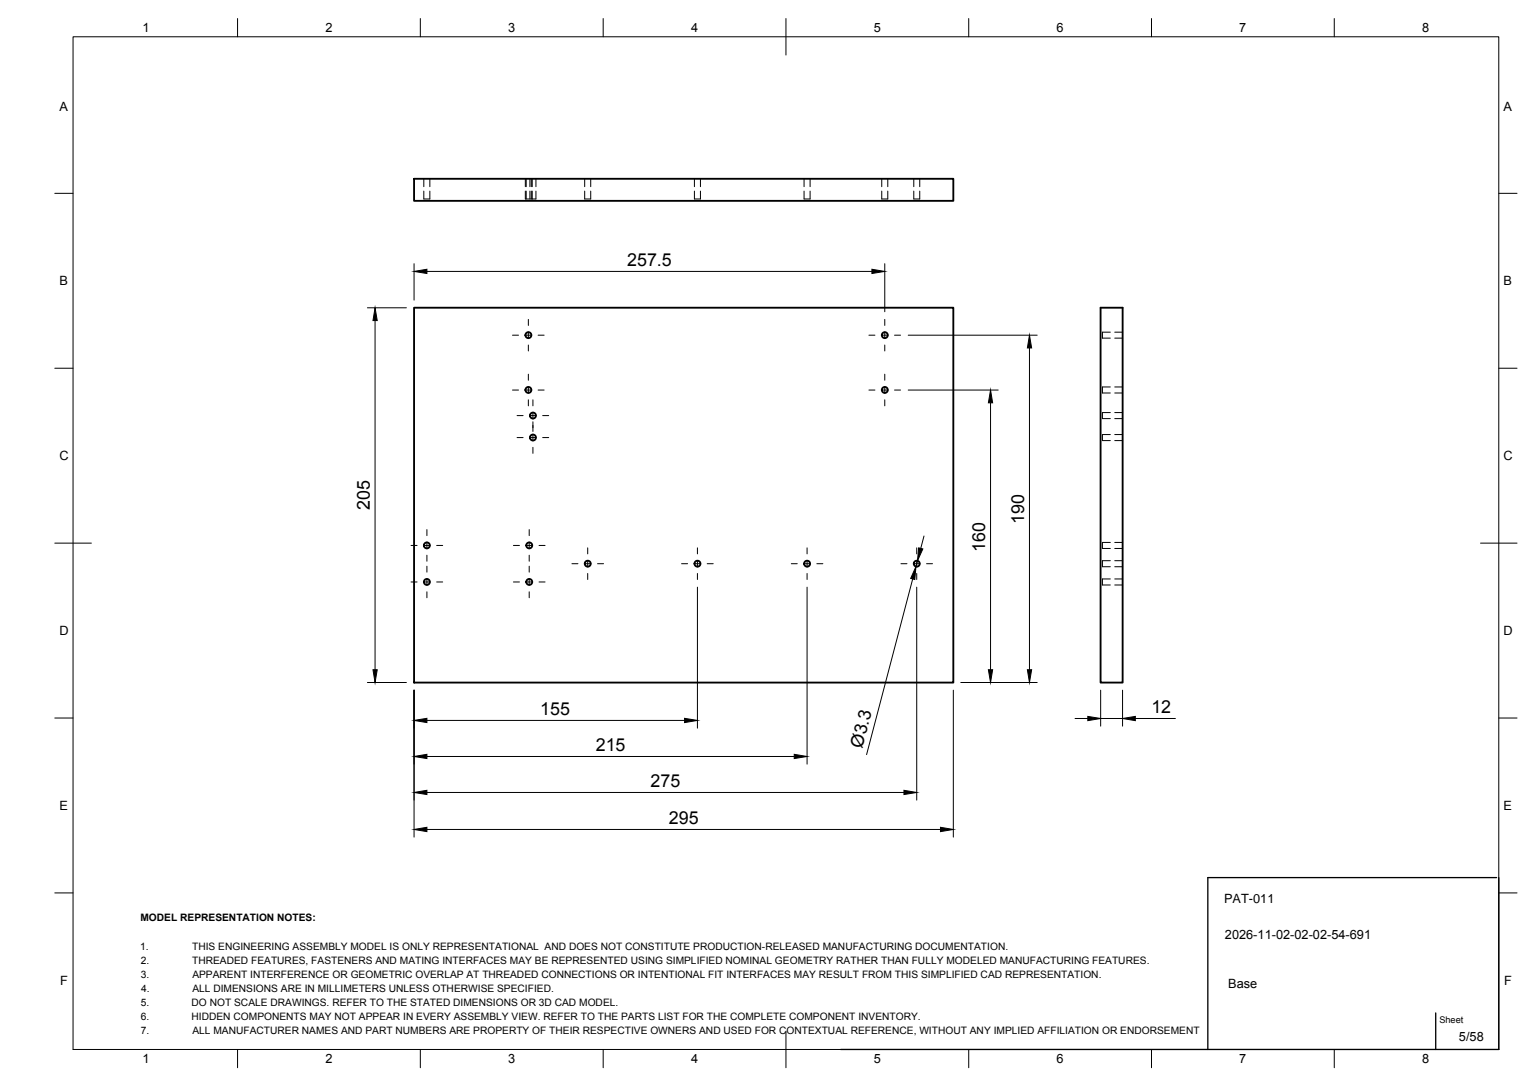
ISO-10303-21;
HEADER;
/* Generated by software containing ST-Developer
 * from STEP Tools, Inc. (www.steptools.com) 
 */

FILE_DESCRIPTION(
/* description */ ('Belt tension measurement rig'),
/* implementation_level */ '2;1');

FILE_NAME(
/* name */ 'Base.step',
/* time_stamp */ '2026-10-28T03:24:44-07:00',
/* author */ (''),
/* organization */ (''),
/* preprocessor_version */ 'ST-DEVELOPER v20.2',
/* originating_system */ 'Autodesk Translation Framework v15.17.0.0',
/* authorisation */ '');

FILE_SCHEMA (('AUTOMOTIVE_DESIGN { 1 0 10303 214 3 1 1 }'));
ENDSEC;

DATA;
#10=MECHANICAL_DESIGN_GEOMETRIC_PRESENTATION_REPRESENTATION('',(#692),#23587);
#582=SHAPE_REPRESENTATION_RELATIONSHIP('SRR','None',#23827,#637);
#637=ADVANCED_BREP_SHAPE_REPRESENTATION('',(#762),#23525);
#692=STYLED_ITEM('',(#24190),#762);
#762=MANIFOLD_SOLID_BREP('Body1',#12197);
#829=FACE_BOUND('',#2089,.T.);
#830=FACE_BOUND('',#2090,.T.);
#831=FACE_BOUND('',#2091,.T.);
#832=FACE_BOUND('',#2092,.T.);
#833=FACE_BOUND('',#2093,.T.);
#834=FACE_BOUND('',#2094,.T.);
#835=FACE_BOUND('',#2095,.T.);
#836=FACE_BOUND('',#2096,.T.);
#837=FACE_BOUND('',#2097,.T.);
#838=FACE_BOUND('',#2098,.T.);
#839=FACE_BOUND('',#2099,.T.);
#840=FACE_BOUND('',#2100,.T.);
#841=FACE_BOUND('',#2101,.T.);
#842=FACE_BOUND('',#2102,.T.);
#1037=PLANE('',#12882);
#1038=PLANE('',#12886);
#1039=PLANE('',#12890);
#1040=PLANE('',#12894);
#1041=PLANE('',#12898);
#1042=PLANE('',#12902);
#1043=PLANE('',#12906);
#1044=PLANE('',#12910);
#1045=PLANE('',#12914);
#1046=PLANE('',#12918);
#1047=PLANE('',#12922);
#1048=PLANE('',#12926);
#1049=PLANE('',#12930);
#1050=PLANE('',#12934);
#1051=PLANE('',#12935);
#1052=PLANE('',#12936);
#1053=PLANE('',#12937);
#1054=PLANE('',#12938);
#1055=PLANE('',#12939);
#1056=PLANE('',#12940);
#1352=FACE_OUTER_BOUND('',#2056,.T.);
#1353=FACE_OUTER_BOUND('',#2057,.T.);
#1354=FACE_OUTER_BOUND('',#2058,.T.);
#1355=FACE_OUTER_BOUND('',#2059,.T.);
#1356=FACE_OUTER_BOUND('',#2060,.T.);
#1357=FACE_OUTER_BOUND('',#2061,.T.);
#1358=FACE_OUTER_BOUND('',#2062,.T.);
#1359=FACE_OUTER_BOUND('',#2063,.T.);
#1360=FACE_OUTER_BOUND('',#2064,.T.);
#1361=FACE_OUTER_BOUND('',#2065,.T.);
#1362=FACE_OUTER_BOUND('',#2066,.T.);
#1363=FACE_OUTER_BOUND('',#2067,.T.);
#1364=FACE_OUTER_BOUND('',#2068,.T.);
#1365=FACE_OUTER_BOUND('',#2069,.T.);
#1366=FACE_OUTER_BOUND('',#2070,.T.);
#1367=FACE_OUTER_BOUND('',#2071,.T.);
#1368=FACE_OUTER_BOUND('',#2072,.T.);
#1369=FACE_OUTER_BOUND('',#2073,.T.);
#1370=FACE_OUTER_BOUND('',#2074,.T.);
#1371=FACE_OUTER_BOUND('',#2075,.T.);
#1372=FACE_OUTER_BOUND('',#2076,.T.);
#1373=FACE_OUTER_BOUND('',#2077,.T.);
#1374=FACE_OUTER_BOUND('',#2078,.T.);
#1375=FACE_OUTER_BOUND('',#2079,.T.);
#1376=FACE_OUTER_BOUND('',#2080,.T.);
#1377=FACE_OUTER_BOUND('',#2081,.T.);
#1378=FACE_OUTER_BOUND('',#2082,.T.);
#1379=FACE_OUTER_BOUND('',#2083,.T.);
#1380=FACE_OUTER_BOUND('',#2084,.T.);
#1381=FACE_OUTER_BOUND('',#2085,.T.);
#1382=FACE_OUTER_BOUND('',#2086,.T.);
#1383=FACE_OUTER_BOUND('',#2087,.T.);
#1384=FACE_OUTER_BOUND('',#2088,.T.);
#1385=FACE_OUTER_BOUND('',#2103,.T.);
#2056=EDGE_LOOP('',(#7938,#7939,#7940,#7941));
#2057=EDGE_LOOP('',(#7942));
#2058=EDGE_LOOP('',(#7943,#7944,#7945,#7946));
#2059=EDGE_LOOP('',(#7947));
#2060=EDGE_LOOP('',(#7948,#7949,#7950,#7951));
#2061=EDGE_LOOP('',(#7952));
#2062=EDGE_LOOP('',(#7953,#7954,#7955,#7956));
#2063=EDGE_LOOP('',(#7957));
#2064=EDGE_LOOP('',(#7958,#7959,#7960,#7961));
#2065=EDGE_LOOP('',(#7962));
#2066=EDGE_LOOP('',(#7963,#7964,#7965,#7966));
#2067=EDGE_LOOP('',(#7967));
#2068=EDGE_LOOP('',(#7968,#7969,#7970,#7971));
#2069=EDGE_LOOP('',(#7972));
#2070=EDGE_LOOP('',(#7973,#7974,#7975,#7976));
#2071=EDGE_LOOP('',(#7977));
#2072=EDGE_LOOP('',(#7978,#7979,#7980,#7981));
#2073=EDGE_LOOP('',(#7982));
#2074=EDGE_LOOP('',(#7983,#7984,#7985,#7986));
#2075=EDGE_LOOP('',(#7987));
#2076=EDGE_LOOP('',(#7988,#7989,#7990,#7991));
#2077=EDGE_LOOP('',(#7992));
#2078=EDGE_LOOP('',(#7993,#7994,#7995,#7996));
#2079=EDGE_LOOP('',(#7997));
#2080=EDGE_LOOP('',(#7998,#7999,#8000,#8001));
#2081=EDGE_LOOP('',(#8002));
#2082=EDGE_LOOP('',(#8003,#8004,#8005,#8006));
#2083=EDGE_LOOP('',(#8007));
#2084=EDGE_LOOP('',(#8008,#8009,#8010,#8011));
#2085=EDGE_LOOP('',(#8012,#8013,#8014,#8015));
#2086=EDGE_LOOP('',(#8016,#8017,#8018,#8019));
#2087=EDGE_LOOP('',(#8020,#8021,#8022,#8023));
#2088=EDGE_LOOP('',(#8024,#8025,#8026,#8027));
#2089=EDGE_LOOP('',(#8028));
#2090=EDGE_LOOP('',(#8029));
#2091=EDGE_LOOP('',(#8030));
#2092=EDGE_LOOP('',(#8031));
#2093=EDGE_LOOP('',(#8032));
#2094=EDGE_LOOP('',(#8033));
#2095=EDGE_LOOP('',(#8034));
#2096=EDGE_LOOP('',(#8035));
#2097=EDGE_LOOP('',(#8036));
#2098=EDGE_LOOP('',(#8037));
#2099=EDGE_LOOP('',(#8038));
#2100=EDGE_LOOP('',(#8039));
#2101=EDGE_LOOP('',(#8040));
#2102=EDGE_LOOP('',(#8041));
#2103=EDGE_LOOP('',(#8042,#8043,#8044,#8045));
#2968=LINE('',#18557,#3719);
#2969=LINE('',#18564,#3720);
#2970=LINE('',#18571,#3721);
#2971=LINE('',#18578,#3722);
#2972=LINE('',#18585,#3723);
#2973=LINE('',#18592,#3724);
#2974=LINE('',#18599,#3725);
#2975=LINE('',#18606,#3726);
#2976=LINE('',#18613,#3727);
#2977=LINE('',#18620,#3728);
#2978=LINE('',#18627,#3729);
#2979=LINE('',#18634,#3730);
#2980=LINE('',#18641,#3731);
#2981=LINE('',#18648,#3732);
#2982=LINE('',#18654,#3733);
#2983=LINE('',#18656,#3734);
#2984=LINE('',#18658,#3735);
#2985=LINE('',#18659,#3736);
#2986=LINE('',#18662,#3737);
#2987=LINE('',#18664,#3738);
#2988=LINE('',#18665,#3739);
#2989=LINE('',#18668,#3740);
#2990=LINE('',#18670,#3741);
#2991=LINE('',#18671,#3742);
#2992=LINE('',#18673,#3743);
#2993=LINE('',#18674,#3744);
#3719=VECTOR('',#14527,0.165);
#3720=VECTOR('',#14536,0.165);
#3721=VECTOR('',#14545,0.164999999999999);
#3722=VECTOR('',#14554,0.164999999999999);
#3723=VECTOR('',#14563,0.165);
#3724=VECTOR('',#14572,0.165);
#3725=VECTOR('',#14581,0.165);
#3726=VECTOR('',#14590,0.165);
#3727=VECTOR('',#14599,0.165);
#3728=VECTOR('',#14608,0.165);
#3729=VECTOR('',#14617,0.164999999999999);
#3730=VECTOR('',#14626,0.164999999999999);
#3731=VECTOR('',#14635,0.165);
#3732=VECTOR('',#14644,0.164999999999999);
#3733=VECTOR('',#14651,1.);
#3734=VECTOR('',#14652,1.);
#3735=VECTOR('',#14653,1.);
#3736=VECTOR('',#14654,1.);
#3737=VECTOR('',#14657,1.);
#3738=VECTOR('',#14658,1.);
#3739=VECTOR('',#14659,1.);
#3740=VECTOR('',#14662,1.);
#3741=VECTOR('',#14663,1.);
#3742=VECTOR('',#14664,1.);
#3743=VECTOR('',#14667,1.);
#3744=VECTOR('',#14668,1.);
#4470=CIRCLE('',#12880,0.165);
#4471=CIRCLE('',#12881,0.165);
#4472=CIRCLE('',#12884,0.165);
#4473=CIRCLE('',#12885,0.165);
#4474=CIRCLE('',#12888,0.164999999999999);
#4475=CIRCLE('',#12889,0.164999999999999);
#4476=CIRCLE('',#12892,0.164999999999999);
#4477=CIRCLE('',#12893,0.164999999999999);
#4478=CIRCLE('',#12896,0.165);
#4479=CIRCLE('',#12897,0.165);
#4480=CIRCLE('',#12900,0.165);
#4481=CIRCLE('',#12901,0.165);
#4482=CIRCLE('',#12904,0.165);
#4483=CIRCLE('',#12905,0.165);
#4484=CIRCLE('',#12908,0.165);
#4485=CIRCLE('',#12909,0.165);
#4486=CIRCLE('',#12912,0.165);
#4487=CIRCLE('',#12913,0.165);
#4488=CIRCLE('',#12916,0.165);
#4489=CIRCLE('',#12917,0.165);
#4490=CIRCLE('',#12920,0.164999999999999);
#4491=CIRCLE('',#12921,0.164999999999999);
#4492=CIRCLE('',#12924,0.164999999999999);
#4493=CIRCLE('',#12925,0.164999999999999);
#4494=CIRCLE('',#12928,0.165);
#4495=CIRCLE('',#12929,0.165);
#4496=CIRCLE('',#12932,0.164999999999999);
#4497=CIRCLE('',#12933,0.164999999999999);
#5238=VERTEX_POINT('',#18554);
#5239=VERTEX_POINT('',#18556);
#5240=VERTEX_POINT('',#18561);
#5241=VERTEX_POINT('',#18563);
#5242=VERTEX_POINT('',#18568);
#5243=VERTEX_POINT('',#18570);
#5244=VERTEX_POINT('',#18575);
#5245=VERTEX_POINT('',#18577);
#5246=VERTEX_POINT('',#18582);
#5247=VERTEX_POINT('',#18584);
#5248=VERTEX_POINT('',#18589);
#5249=VERTEX_POINT('',#18591);
#5250=VERTEX_POINT('',#18596);
#5251=VERTEX_POINT('',#18598);
#5252=VERTEX_POINT('',#18603);
#5253=VERTEX_POINT('',#18605);
#5254=VERTEX_POINT('',#18610);
#5255=VERTEX_POINT('',#18612);
#5256=VERTEX_POINT('',#18617);
#5257=VERTEX_POINT('',#18619);
#5258=VERTEX_POINT('',#18624);
#5259=VERTEX_POINT('',#18626);
#5260=VERTEX_POINT('',#18631);
#5261=VERTEX_POINT('',#18633);
#5262=VERTEX_POINT('',#18638);
#5263=VERTEX_POINT('',#18640);
#5264=VERTEX_POINT('',#18645);
#5265=VERTEX_POINT('',#18647);
#5266=VERTEX_POINT('',#18652);
#5267=VERTEX_POINT('',#18653);
#5268=VERTEX_POINT('',#18655);
#5269=VERTEX_POINT('',#18657);
#5270=VERTEX_POINT('',#18661);
#5271=VERTEX_POINT('',#18663);
#5272=VERTEX_POINT('',#18667);
#5273=VERTEX_POINT('',#18669);
#6328=EDGE_CURVE('',#5238,#5238,#4470,.T.);
#6329=EDGE_CURVE('',#5238,#5239,#2968,.T.);
#6330=EDGE_CURVE('',#5239,#5239,#4471,.T.);
#6331=EDGE_CURVE('',#5240,#5240,#4472,.T.);
#6332=EDGE_CURVE('',#5240,#5241,#2969,.T.);
#6333=EDGE_CURVE('',#5241,#5241,#4473,.T.);
#6334=EDGE_CURVE('',#5242,#5242,#4474,.T.);
#6335=EDGE_CURVE('',#5242,#5243,#2970,.T.);
#6336=EDGE_CURVE('',#5243,#5243,#4475,.T.);
#6337=EDGE_CURVE('',#5244,#5244,#4476,.T.);
#6338=EDGE_CURVE('',#5244,#5245,#2971,.T.);
#6339=EDGE_CURVE('',#5245,#5245,#4477,.T.);
#6340=EDGE_CURVE('',#5246,#5246,#4478,.T.);
#6341=EDGE_CURVE('',#5246,#5247,#2972,.T.);
#6342=EDGE_CURVE('',#5247,#5247,#4479,.T.);
#6343=EDGE_CURVE('',#5248,#5248,#4480,.T.);
#6344=EDGE_CURVE('',#5248,#5249,#2973,.T.);
#6345=EDGE_CURVE('',#5249,#5249,#4481,.T.);
#6346=EDGE_CURVE('',#5250,#5250,#4482,.T.);
#6347=EDGE_CURVE('',#5250,#5251,#2974,.T.);
#6348=EDGE_CURVE('',#5251,#5251,#4483,.T.);
#6349=EDGE_CURVE('',#5252,#5252,#4484,.T.);
#6350=EDGE_CURVE('',#5252,#5253,#2975,.T.);
#6351=EDGE_CURVE('',#5253,#5253,#4485,.T.);
#6352=EDGE_CURVE('',#5254,#5254,#4486,.T.);
#6353=EDGE_CURVE('',#5254,#5255,#2976,.T.);
#6354=EDGE_CURVE('',#5255,#5255,#4487,.T.);
#6355=EDGE_CURVE('',#5256,#5256,#4488,.T.);
#6356=EDGE_CURVE('',#5256,#5257,#2977,.T.);
#6357=EDGE_CURVE('',#5257,#5257,#4489,.T.);
#6358=EDGE_CURVE('',#5258,#5258,#4490,.T.);
#6359=EDGE_CURVE('',#5258,#5259,#2978,.T.);
#6360=EDGE_CURVE('',#5259,#5259,#4491,.T.);
#6361=EDGE_CURVE('',#5260,#5260,#4492,.T.);
#6362=EDGE_CURVE('',#5260,#5261,#2979,.T.);
#6363=EDGE_CURVE('',#5261,#5261,#4493,.T.);
#6364=EDGE_CURVE('',#5262,#5262,#4494,.T.);
#6365=EDGE_CURVE('',#5262,#5263,#2980,.T.);
#6366=EDGE_CURVE('',#5263,#5263,#4495,.T.);
#6367=EDGE_CURVE('',#5264,#5264,#4496,.T.);
#6368=EDGE_CURVE('',#5264,#5265,#2981,.T.);
#6369=EDGE_CURVE('',#5265,#5265,#4497,.T.);
#6370=EDGE_CURVE('',#5266,#5267,#2982,.T.);
#6371=EDGE_CURVE('',#5267,#5268,#2983,.T.);
#6372=EDGE_CURVE('',#5269,#5268,#2984,.T.);
#6373=EDGE_CURVE('',#5266,#5269,#2985,.T.);
#6374=EDGE_CURVE('',#5270,#5266,#2986,.T.);
#6375=EDGE_CURVE('',#5271,#5269,#2987,.T.);
#6376=EDGE_CURVE('',#5270,#5271,#2988,.T.);
#6377=EDGE_CURVE('',#5272,#5270,#2989,.T.);
#6378=EDGE_CURVE('',#5273,#5271,#2990,.T.);
#6379=EDGE_CURVE('',#5272,#5273,#2991,.T.);
#6380=EDGE_CURVE('',#5267,#5272,#2992,.T.);
#6381=EDGE_CURVE('',#5268,#5273,#2993,.T.);
#7938=ORIENTED_EDGE('',*,*,#6328,.F.);
#7939=ORIENTED_EDGE('',*,*,#6329,.T.);
#7940=ORIENTED_EDGE('',*,*,#6330,.F.);
#7941=ORIENTED_EDGE('',*,*,#6329,.F.);
#7942=ORIENTED_EDGE('',*,*,#6328,.T.);
#7943=ORIENTED_EDGE('',*,*,#6331,.F.);
#7944=ORIENTED_EDGE('',*,*,#6332,.T.);
#7945=ORIENTED_EDGE('',*,*,#6333,.F.);
#7946=ORIENTED_EDGE('',*,*,#6332,.F.);
#7947=ORIENTED_EDGE('',*,*,#6331,.T.);
#7948=ORIENTED_EDGE('',*,*,#6334,.F.);
#7949=ORIENTED_EDGE('',*,*,#6335,.T.);
#7950=ORIENTED_EDGE('',*,*,#6336,.F.);
#7951=ORIENTED_EDGE('',*,*,#6335,.F.);
#7952=ORIENTED_EDGE('',*,*,#6334,.T.);
#7953=ORIENTED_EDGE('',*,*,#6337,.F.);
#7954=ORIENTED_EDGE('',*,*,#6338,.T.);
#7955=ORIENTED_EDGE('',*,*,#6339,.F.);
#7956=ORIENTED_EDGE('',*,*,#6338,.F.);
#7957=ORIENTED_EDGE('',*,*,#6337,.T.);
#7958=ORIENTED_EDGE('',*,*,#6340,.F.);
#7959=ORIENTED_EDGE('',*,*,#6341,.T.);
#7960=ORIENTED_EDGE('',*,*,#6342,.F.);
#7961=ORIENTED_EDGE('',*,*,#6341,.F.);
#7962=ORIENTED_EDGE('',*,*,#6340,.T.);
#7963=ORIENTED_EDGE('',*,*,#6343,.F.);
#7964=ORIENTED_EDGE('',*,*,#6344,.T.);
#7965=ORIENTED_EDGE('',*,*,#6345,.F.);
#7966=ORIENTED_EDGE('',*,*,#6344,.F.);
#7967=ORIENTED_EDGE('',*,*,#6343,.T.);
#7968=ORIENTED_EDGE('',*,*,#6346,.F.);
#7969=ORIENTED_EDGE('',*,*,#6347,.T.);
#7970=ORIENTED_EDGE('',*,*,#6348,.F.);
#7971=ORIENTED_EDGE('',*,*,#6347,.F.);
#7972=ORIENTED_EDGE('',*,*,#6346,.T.);
#7973=ORIENTED_EDGE('',*,*,#6349,.F.);
#7974=ORIENTED_EDGE('',*,*,#6350,.T.);
#7975=ORIENTED_EDGE('',*,*,#6351,.F.);
#7976=ORIENTED_EDGE('',*,*,#6350,.F.);
#7977=ORIENTED_EDGE('',*,*,#6349,.T.);
#7978=ORIENTED_EDGE('',*,*,#6352,.F.);
#7979=ORIENTED_EDGE('',*,*,#6353,.T.);
#7980=ORIENTED_EDGE('',*,*,#6354,.F.);
#7981=ORIENTED_EDGE('',*,*,#6353,.F.);
#7982=ORIENTED_EDGE('',*,*,#6352,.T.);
#7983=ORIENTED_EDGE('',*,*,#6355,.F.);
#7984=ORIENTED_EDGE('',*,*,#6356,.T.);
#7985=ORIENTED_EDGE('',*,*,#6357,.F.);
#7986=ORIENTED_EDGE('',*,*,#6356,.F.);
#7987=ORIENTED_EDGE('',*,*,#6355,.T.);
#7988=ORIENTED_EDGE('',*,*,#6358,.F.);
#7989=ORIENTED_EDGE('',*,*,#6359,.T.);
#7990=ORIENTED_EDGE('',*,*,#6360,.F.);
#7991=ORIENTED_EDGE('',*,*,#6359,.F.);
#7992=ORIENTED_EDGE('',*,*,#6358,.T.);
#7993=ORIENTED_EDGE('',*,*,#6361,.F.);
#7994=ORIENTED_EDGE('',*,*,#6362,.T.);
#7995=ORIENTED_EDGE('',*,*,#6363,.F.);
#7996=ORIENTED_EDGE('',*,*,#6362,.F.);
#7997=ORIENTED_EDGE('',*,*,#6361,.T.);
#7998=ORIENTED_EDGE('',*,*,#6364,.F.);
#7999=ORIENTED_EDGE('',*,*,#6365,.T.);
#8000=ORIENTED_EDGE('',*,*,#6366,.F.);
#8001=ORIENTED_EDGE('',*,*,#6365,.F.);
#8002=ORIENTED_EDGE('',*,*,#6364,.T.);
#8003=ORIENTED_EDGE('',*,*,#6367,.F.);
#8004=ORIENTED_EDGE('',*,*,#6368,.T.);
#8005=ORIENTED_EDGE('',*,*,#6369,.F.);
#8006=ORIENTED_EDGE('',*,*,#6368,.F.);
#8007=ORIENTED_EDGE('',*,*,#6367,.T.);
#8008=ORIENTED_EDGE('',*,*,#6370,.T.);
#8009=ORIENTED_EDGE('',*,*,#6371,.T.);
#8010=ORIENTED_EDGE('',*,*,#6372,.F.);
#8011=ORIENTED_EDGE('',*,*,#6373,.F.);
#8012=ORIENTED_EDGE('',*,*,#6374,.T.);
#8013=ORIENTED_EDGE('',*,*,#6373,.T.);
#8014=ORIENTED_EDGE('',*,*,#6375,.F.);
#8015=ORIENTED_EDGE('',*,*,#6376,.F.);
#8016=ORIENTED_EDGE('',*,*,#6377,.T.);
#8017=ORIENTED_EDGE('',*,*,#6376,.T.);
#8018=ORIENTED_EDGE('',*,*,#6378,.F.);
#8019=ORIENTED_EDGE('',*,*,#6379,.F.);
#8020=ORIENTED_EDGE('',*,*,#6380,.T.);
#8021=ORIENTED_EDGE('',*,*,#6379,.T.);
#8022=ORIENTED_EDGE('',*,*,#6381,.F.);
#8023=ORIENTED_EDGE('',*,*,#6371,.F.);
#8024=ORIENTED_EDGE('',*,*,#6381,.T.);
#8025=ORIENTED_EDGE('',*,*,#6378,.T.);
#8026=ORIENTED_EDGE('',*,*,#6375,.T.);
#8027=ORIENTED_EDGE('',*,*,#6372,.T.);
#8028=ORIENTED_EDGE('',*,*,#6336,.T.);
#8029=ORIENTED_EDGE('',*,*,#6339,.T.);
#8030=ORIENTED_EDGE('',*,*,#6348,.T.);
#8031=ORIENTED_EDGE('',*,*,#6351,.T.);
#8032=ORIENTED_EDGE('',*,*,#6354,.T.);
#8033=ORIENTED_EDGE('',*,*,#6357,.T.);
#8034=ORIENTED_EDGE('',*,*,#6360,.T.);
#8035=ORIENTED_EDGE('',*,*,#6363,.T.);
#8036=ORIENTED_EDGE('',*,*,#6366,.T.);
#8037=ORIENTED_EDGE('',*,*,#6369,.T.);
#8038=ORIENTED_EDGE('',*,*,#6345,.T.);
#8039=ORIENTED_EDGE('',*,*,#6342,.T.);
#8040=ORIENTED_EDGE('',*,*,#6333,.T.);
#8041=ORIENTED_EDGE('',*,*,#6330,.T.);
#8042=ORIENTED_EDGE('',*,*,#6380,.F.);
#8043=ORIENTED_EDGE('',*,*,#6370,.F.);
#8044=ORIENTED_EDGE('',*,*,#6374,.F.);
#8045=ORIENTED_EDGE('',*,*,#6377,.F.);
#11158=CYLINDRICAL_SURFACE('',#12879,0.165);
#11159=CYLINDRICAL_SURFACE('',#12883,0.165);
#11160=CYLINDRICAL_SURFACE('',#12887,0.164999999999999);
#11161=CYLINDRICAL_SURFACE('',#12891,0.164999999999999);
#11162=CYLINDRICAL_SURFACE('',#12895,0.165);
#11163=CYLINDRICAL_SURFACE('',#12899,0.165);
#11164=CYLINDRICAL_SURFACE('',#12903,0.165);
#11165=CYLINDRICAL_SURFACE('',#12907,0.165);
#11166=CYLINDRICAL_SURFACE('',#12911,0.165);
#11167=CYLINDRICAL_SURFACE('',#12915,0.165);
#11168=CYLINDRICAL_SURFACE('',#12919,0.164999999999999);
#11169=CYLINDRICAL_SURFACE('',#12923,0.164999999999999);
#11170=CYLINDRICAL_SURFACE('',#12927,0.165);
#11171=CYLINDRICAL_SURFACE('',#12931,0.164999999999999);
#11493=ADVANCED_FACE('',(#1352),#11158,.F.);
#11494=ADVANCED_FACE('',(#1353),#1037,.T.);
#11495=ADVANCED_FACE('',(#1354),#11159,.F.);
#11496=ADVANCED_FACE('',(#1355),#1038,.T.);
#11497=ADVANCED_FACE('',(#1356),#11160,.F.);
#11498=ADVANCED_FACE('',(#1357),#1039,.T.);
#11499=ADVANCED_FACE('',(#1358),#11161,.F.);
#11500=ADVANCED_FACE('',(#1359),#1040,.T.);
#11501=ADVANCED_FACE('',(#1360),#11162,.F.);
#11502=ADVANCED_FACE('',(#1361),#1041,.T.);
#11503=ADVANCED_FACE('',(#1362),#11163,.F.);
#11504=ADVANCED_FACE('',(#1363),#1042,.T.);
#11505=ADVANCED_FACE('',(#1364),#11164,.F.);
#11506=ADVANCED_FACE('',(#1365),#1043,.T.);
#11507=ADVANCED_FACE('',(#1366),#11165,.F.);
#11508=ADVANCED_FACE('',(#1367),#1044,.T.);
#11509=ADVANCED_FACE('',(#1368),#11166,.F.);
#11510=ADVANCED_FACE('',(#1369),#1045,.T.);
#11511=ADVANCED_FACE('',(#1370),#11167,.F.);
#11512=ADVANCED_FACE('',(#1371),#1046,.T.);
#11513=ADVANCED_FACE('',(#1372),#11168,.F.);
#11514=ADVANCED_FACE('',(#1373),#1047,.T.);
#11515=ADVANCED_FACE('',(#1374),#11169,.F.);
#11516=ADVANCED_FACE('',(#1375),#1048,.T.);
#11517=ADVANCED_FACE('',(#1376),#11170,.F.);
#11518=ADVANCED_FACE('',(#1377),#1049,.T.);
#11519=ADVANCED_FACE('',(#1378),#11171,.F.);
#11520=ADVANCED_FACE('',(#1379),#1050,.T.);
#11521=ADVANCED_FACE('',(#1380),#1051,.T.);
#11522=ADVANCED_FACE('',(#1381),#1052,.T.);
#11523=ADVANCED_FACE('',(#1382),#1053,.T.);
#11524=ADVANCED_FACE('',(#1383),#1054,.T.);
#11525=ADVANCED_FACE('',(#1384,#829,#830,#831,#832,#833,#834,#835,#836,
#837,#838,#839,#840,#841,#842),#1055,.T.);
#11526=ADVANCED_FACE('',(#1385),#1056,.F.);
#12197=CLOSED_SHELL('',(#11493,#11494,#11495,#11496,#11497,#11498,#11499,
#11500,#11501,#11502,#11503,#11504,#11505,#11506,#11507,#11508,#11509,#11510,
#11511,#11512,#11513,#11514,#11515,#11516,#11517,#11518,#11519,#11520,#11521,
#11522,#11523,#11524,#11525,#11526));
#12878=AXIS2_PLACEMENT_3D('',#18552,#14521,#14522);
#12879=AXIS2_PLACEMENT_3D('',#18553,#14523,#14524);
#12880=AXIS2_PLACEMENT_3D('',#18555,#14525,#14526);
#12881=AXIS2_PLACEMENT_3D('',#18558,#14528,#14529);
#12882=AXIS2_PLACEMENT_3D('',#18559,#14530,#14531);
#12883=AXIS2_PLACEMENT_3D('',#18560,#14532,#14533);
#12884=AXIS2_PLACEMENT_3D('',#18562,#14534,#14535);
#12885=AXIS2_PLACEMENT_3D('',#18565,#14537,#14538);
#12886=AXIS2_PLACEMENT_3D('',#18566,#14539,#14540);
#12887=AXIS2_PLACEMENT_3D('',#18567,#14541,#14542);
#12888=AXIS2_PLACEMENT_3D('',#18569,#14543,#14544);
#12889=AXIS2_PLACEMENT_3D('',#18572,#14546,#14547);
#12890=AXIS2_PLACEMENT_3D('',#18573,#14548,#14549);
#12891=AXIS2_PLACEMENT_3D('',#18574,#14550,#14551);
#12892=AXIS2_PLACEMENT_3D('',#18576,#14552,#14553);
#12893=AXIS2_PLACEMENT_3D('',#18579,#14555,#14556);
#12894=AXIS2_PLACEMENT_3D('',#18580,#14557,#14558);
#12895=AXIS2_PLACEMENT_3D('',#18581,#14559,#14560);
#12896=AXIS2_PLACEMENT_3D('',#18583,#14561,#14562);
#12897=AXIS2_PLACEMENT_3D('',#18586,#14564,#14565);
#12898=AXIS2_PLACEMENT_3D('',#18587,#14566,#14567);
#12899=AXIS2_PLACEMENT_3D('',#18588,#14568,#14569);
#12900=AXIS2_PLACEMENT_3D('',#18590,#14570,#14571);
#12901=AXIS2_PLACEMENT_3D('',#18593,#14573,#14574);
#12902=AXIS2_PLACEMENT_3D('',#18594,#14575,#14576);
#12903=AXIS2_PLACEMENT_3D('',#18595,#14577,#14578);
#12904=AXIS2_PLACEMENT_3D('',#18597,#14579,#14580);
#12905=AXIS2_PLACEMENT_3D('',#18600,#14582,#14583);
#12906=AXIS2_PLACEMENT_3D('',#18601,#14584,#14585);
#12907=AXIS2_PLACEMENT_3D('',#18602,#14586,#14587);
#12908=AXIS2_PLACEMENT_3D('',#18604,#14588,#14589);
#12909=AXIS2_PLACEMENT_3D('',#18607,#14591,#14592);
#12910=AXIS2_PLACEMENT_3D('',#18608,#14593,#14594);
#12911=AXIS2_PLACEMENT_3D('',#18609,#14595,#14596);
#12912=AXIS2_PLACEMENT_3D('',#18611,#14597,#14598);
#12913=AXIS2_PLACEMENT_3D('',#18614,#14600,#14601);
#12914=AXIS2_PLACEMENT_3D('',#18615,#14602,#14603);
#12915=AXIS2_PLACEMENT_3D('',#18616,#14604,#14605);
#12916=AXIS2_PLACEMENT_3D('',#18618,#14606,#14607);
#12917=AXIS2_PLACEMENT_3D('',#18621,#14609,#14610);
#12918=AXIS2_PLACEMENT_3D('',#18622,#14611,#14612);
#12919=AXIS2_PLACEMENT_3D('',#18623,#14613,#14614);
#12920=AXIS2_PLACEMENT_3D('',#18625,#14615,#14616);
#12921=AXIS2_PLACEMENT_3D('',#18628,#14618,#14619);
#12922=AXIS2_PLACEMENT_3D('',#18629,#14620,#14621);
#12923=AXIS2_PLACEMENT_3D('',#18630,#14622,#14623);
#12924=AXIS2_PLACEMENT_3D('',#18632,#14624,#14625);
#12925=AXIS2_PLACEMENT_3D('',#18635,#14627,#14628);
#12926=AXIS2_PLACEMENT_3D('',#18636,#14629,#14630);
#12927=AXIS2_PLACEMENT_3D('',#18637,#14631,#14632);
#12928=AXIS2_PLACEMENT_3D('',#18639,#14633,#14634);
#12929=AXIS2_PLACEMENT_3D('',#18642,#14636,#14637);
#12930=AXIS2_PLACEMENT_3D('',#18643,#14638,#14639);
#12931=AXIS2_PLACEMENT_3D('',#18644,#14640,#14641);
#12932=AXIS2_PLACEMENT_3D('',#18646,#14642,#14643);
#12933=AXIS2_PLACEMENT_3D('',#18649,#14645,#14646);
#12934=AXIS2_PLACEMENT_3D('',#18650,#14647,#14648);
#12935=AXIS2_PLACEMENT_3D('',#18651,#14649,#14650);
#12936=AXIS2_PLACEMENT_3D('',#18660,#14655,#14656);
#12937=AXIS2_PLACEMENT_3D('',#18666,#14660,#14661);
#12938=AXIS2_PLACEMENT_3D('',#18672,#14665,#14666);
#12939=AXIS2_PLACEMENT_3D('',#18675,#14669,#14670);
#12940=AXIS2_PLACEMENT_3D('',#18676,#14671,#14672);
#14521=DIRECTION('axis',(0.,0.,1.));
#14522=DIRECTION('refdir',(1.,0.,0.));
#14523=DIRECTION('center_axis',(0.,0.,1.));
#14524=DIRECTION('ref_axis',(1.,0.,0.));
#14525=DIRECTION('center_axis',(0.,0.,1.));
#14526=DIRECTION('ref_axis',(1.,0.,0.));
#14527=DIRECTION('',(0.,0.,1.));
#14528=DIRECTION('center_axis',(0.,0.,-1.));
#14529=DIRECTION('ref_axis',(1.,0.,0.));
#14530=DIRECTION('center_axis',(0.,0.,1.));
#14531=DIRECTION('ref_axis',(1.,0.,0.));
#14532=DIRECTION('center_axis',(0.,0.,1.));
#14533=DIRECTION('ref_axis',(1.,0.,0.));
#14534=DIRECTION('center_axis',(0.,0.,1.));
#14535=DIRECTION('ref_axis',(1.,0.,0.));
#14536=DIRECTION('',(0.,0.,1.));
#14537=DIRECTION('center_axis',(0.,0.,-1.));
#14538=DIRECTION('ref_axis',(1.,0.,0.));
#14539=DIRECTION('center_axis',(0.,0.,1.));
#14540=DIRECTION('ref_axis',(1.,0.,0.));
#14541=DIRECTION('center_axis',(0.,0.,1.));
#14542=DIRECTION('ref_axis',(1.,0.,0.));
#14543=DIRECTION('center_axis',(0.,0.,1.));
#14544=DIRECTION('ref_axis',(1.,0.,0.));
#14545=DIRECTION('',(0.,0.,1.));
#14546=DIRECTION('center_axis',(0.,0.,-1.));
#14547=DIRECTION('ref_axis',(1.,0.,0.));
#14548=DIRECTION('center_axis',(0.,0.,1.));
#14549=DIRECTION('ref_axis',(1.,0.,0.));
#14550=DIRECTION('center_axis',(0.,0.,1.));
#14551=DIRECTION('ref_axis',(1.,0.,0.));
#14552=DIRECTION('center_axis',(0.,0.,1.));
#14553=DIRECTION('ref_axis',(1.,0.,0.));
#14554=DIRECTION('',(0.,0.,1.));
#14555=DIRECTION('center_axis',(0.,0.,-1.));
#14556=DIRECTION('ref_axis',(1.,0.,0.));
#14557=DIRECTION('center_axis',(0.,0.,1.));
#14558=DIRECTION('ref_axis',(1.,0.,0.));
#14559=DIRECTION('center_axis',(0.,0.,1.));
#14560=DIRECTION('ref_axis',(1.,0.,0.));
#14561=DIRECTION('center_axis',(0.,0.,1.));
#14562=DIRECTION('ref_axis',(1.,0.,0.));
#14563=DIRECTION('',(0.,0.,1.));
#14564=DIRECTION('center_axis',(0.,0.,-1.));
#14565=DIRECTION('ref_axis',(1.,0.,0.));
#14566=DIRECTION('center_axis',(0.,0.,1.));
#14567=DIRECTION('ref_axis',(1.,0.,0.));
#14568=DIRECTION('center_axis',(0.,0.,1.));
#14569=DIRECTION('ref_axis',(1.,0.,0.));
#14570=DIRECTION('center_axis',(0.,0.,1.));
#14571=DIRECTION('ref_axis',(1.,0.,0.));
#14572=DIRECTION('',(0.,0.,1.));
#14573=DIRECTION('center_axis',(0.,0.,-1.));
#14574=DIRECTION('ref_axis',(1.,0.,0.));
#14575=DIRECTION('center_axis',(0.,0.,1.));
#14576=DIRECTION('ref_axis',(1.,0.,0.));
#14577=DIRECTION('center_axis',(0.,0.,1.));
#14578=DIRECTION('ref_axis',(1.,0.,0.));
#14579=DIRECTION('center_axis',(0.,0.,1.));
#14580=DIRECTION('ref_axis',(1.,0.,0.));
#14581=DIRECTION('',(0.,0.,1.));
#14582=DIRECTION('center_axis',(0.,0.,-1.));
#14583=DIRECTION('ref_axis',(1.,0.,0.));
#14584=DIRECTION('center_axis',(0.,0.,1.));
#14585=DIRECTION('ref_axis',(1.,0.,0.));
#14586=DIRECTION('center_axis',(0.,0.,1.));
#14587=DIRECTION('ref_axis',(1.,0.,0.));
#14588=DIRECTION('center_axis',(0.,0.,1.));
#14589=DIRECTION('ref_axis',(1.,0.,0.));
#14590=DIRECTION('',(0.,0.,1.));
#14591=DIRECTION('center_axis',(0.,0.,-1.));
#14592=DIRECTION('ref_axis',(1.,0.,0.));
#14593=DIRECTION('center_axis',(0.,0.,1.));
#14594=DIRECTION('ref_axis',(1.,0.,0.));
#14595=DIRECTION('center_axis',(0.,0.,1.));
#14596=DIRECTION('ref_axis',(1.,0.,0.));
#14597=DIRECTION('center_axis',(0.,0.,1.));
#14598=DIRECTION('ref_axis',(1.,0.,0.));
#14599=DIRECTION('',(0.,0.,1.));
#14600=DIRECTION('center_axis',(0.,0.,-1.));
#14601=DIRECTION('ref_axis',(1.,0.,0.));
#14602=DIRECTION('center_axis',(0.,0.,1.));
#14603=DIRECTION('ref_axis',(1.,0.,0.));
#14604=DIRECTION('center_axis',(0.,0.,1.));
#14605=DIRECTION('ref_axis',(1.,0.,0.));
#14606=DIRECTION('center_axis',(0.,0.,1.));
#14607=DIRECTION('ref_axis',(1.,0.,0.));
#14608=DIRECTION('',(0.,0.,1.));
#14609=DIRECTION('center_axis',(0.,0.,-1.));
#14610=DIRECTION('ref_axis',(1.,0.,0.));
#14611=DIRECTION('center_axis',(0.,0.,1.));
#14612=DIRECTION('ref_axis',(1.,0.,0.));
#14613=DIRECTION('center_axis',(0.,0.,1.));
#14614=DIRECTION('ref_axis',(1.,0.,0.));
#14615=DIRECTION('center_axis',(0.,0.,1.));
#14616=DIRECTION('ref_axis',(1.,0.,0.));
#14617=DIRECTION('',(0.,0.,1.));
#14618=DIRECTION('center_axis',(0.,0.,-1.));
#14619=DIRECTION('ref_axis',(1.,0.,0.));
#14620=DIRECTION('center_axis',(0.,0.,1.));
#14621=DIRECTION('ref_axis',(1.,0.,0.));
#14622=DIRECTION('center_axis',(0.,0.,1.));
#14623=DIRECTION('ref_axis',(1.,0.,0.));
#14624=DIRECTION('center_axis',(0.,0.,1.));
#14625=DIRECTION('ref_axis',(1.,0.,0.));
#14626=DIRECTION('',(0.,0.,1.));
#14627=DIRECTION('center_axis',(0.,0.,-1.));
#14628=DIRECTION('ref_axis',(1.,0.,0.));
#14629=DIRECTION('center_axis',(0.,0.,1.));
#14630=DIRECTION('ref_axis',(1.,0.,0.));
#14631=DIRECTION('center_axis',(0.,0.,1.));
#14632=DIRECTION('ref_axis',(1.,0.,0.));
#14633=DIRECTION('center_axis',(0.,0.,1.));
#14634=DIRECTION('ref_axis',(1.,0.,0.));
#14635=DIRECTION('',(0.,0.,1.));
#14636=DIRECTION('center_axis',(0.,0.,-1.));
#14637=DIRECTION('ref_axis',(1.,0.,0.));
#14638=DIRECTION('center_axis',(0.,0.,1.));
#14639=DIRECTION('ref_axis',(1.,0.,0.));
#14640=DIRECTION('center_axis',(0.,0.,1.));
#14641=DIRECTION('ref_axis',(1.,0.,0.));
#14642=DIRECTION('center_axis',(0.,0.,1.));
#14643=DIRECTION('ref_axis',(1.,0.,0.));
#14644=DIRECTION('',(0.,0.,1.));
#14645=DIRECTION('center_axis',(0.,0.,-1.));
#14646=DIRECTION('ref_axis',(1.,0.,0.));
#14647=DIRECTION('center_axis',(0.,0.,1.));
#14648=DIRECTION('ref_axis',(1.,0.,0.));
#14649=DIRECTION('center_axis',(0.,1.,0.));
#14650=DIRECTION('ref_axis',(-1.,0.,0.));
#14651=DIRECTION('',(-1.,0.,0.));
#14652=DIRECTION('',(0.,0.,1.));
#14653=DIRECTION('',(-1.,0.,0.));
#14654=DIRECTION('',(0.,0.,1.));
#14655=DIRECTION('center_axis',(1.,0.,0.));
#14656=DIRECTION('ref_axis',(0.,1.,0.));
#14657=DIRECTION('',(0.,1.,0.));
#14658=DIRECTION('',(0.,1.,0.));
#14659=DIRECTION('',(0.,0.,1.));
#14660=DIRECTION('center_axis',(0.,-1.,0.));
#14661=DIRECTION('ref_axis',(1.,0.,0.));
#14662=DIRECTION('',(1.,0.,0.));
#14663=DIRECTION('',(1.,0.,0.));
#14664=DIRECTION('',(0.,0.,1.));
#14665=DIRECTION('center_axis',(-1.,0.,0.));
#14666=DIRECTION('ref_axis',(0.,-1.,0.));
#14667=DIRECTION('',(0.,-1.,0.));
#14668=DIRECTION('',(0.,-1.,0.));
#14669=DIRECTION('center_axis',(0.,0.,1.));
#14670=DIRECTION('ref_axis',(1.,0.,0.));
#14671=DIRECTION('center_axis',(0.,0.,1.));
#14672=DIRECTION('ref_axis',(1.,0.,0.));
#18552=CARTESIAN_POINT('',(0.,0.,0.));
#18553=CARTESIAN_POINT('Origin',(3.,6.9,-1.1));
#18554=CARTESIAN_POINT('',(2.835,6.9,-1.1));
#18555=CARTESIAN_POINT('Origin',(3.,6.9,-1.1));
#18556=CARTESIAN_POINT('',(2.835,6.9,0.));
#18557=CARTESIAN_POINT('',(2.835,6.9,-1.1));
#18558=CARTESIAN_POINT('Origin',(3.,6.9,0.));
#18559=CARTESIAN_POINT('Origin',(3.,6.9,-1.1));
#18560=CARTESIAN_POINT('Origin',(3.,8.1,-1.1));
#18561=CARTESIAN_POINT('',(2.835,8.1,-1.1));
#18562=CARTESIAN_POINT('Origin',(3.,8.1,-1.1));
#18563=CARTESIAN_POINT('',(2.835,8.1,0.));
#18564=CARTESIAN_POINT('',(2.835,8.1,-1.1));
#18565=CARTESIAN_POINT('Origin',(3.,8.1,0.));
#18566=CARTESIAN_POINT('Origin',(3.,8.1,-1.1));
#18567=CARTESIAN_POINT('Origin',(22.25,9.5,-1.1));
#18568=CARTESIAN_POINT('',(22.085,9.5,-1.1));
#18569=CARTESIAN_POINT('Origin',(22.25,9.5,-1.1));
#18570=CARTESIAN_POINT('',(22.085,9.5,0.));
#18571=CARTESIAN_POINT('',(22.085,9.5,-1.1));
#18572=CARTESIAN_POINT('Origin',(22.25,9.5,0.));
#18573=CARTESIAN_POINT('Origin',(22.25,9.5,-1.1));
#18574=CARTESIAN_POINT('Origin',(22.25,12.5,-1.1));
#18575=CARTESIAN_POINT('',(22.085,12.5,-1.1));
#18576=CARTESIAN_POINT('Origin',(22.25,12.5,-1.1));
#18577=CARTESIAN_POINT('',(22.085,12.5,0.));
#18578=CARTESIAN_POINT('',(22.085,12.5,-1.1));
#18579=CARTESIAN_POINT('Origin',(22.25,12.5,0.));
#18580=CARTESIAN_POINT('Origin',(22.25,12.5,-1.1));
#18581=CARTESIAN_POINT('Origin',(2.75,9.5,-1.1));
#18582=CARTESIAN_POINT('',(2.585,9.5,-1.1));
#18583=CARTESIAN_POINT('Origin',(2.75,9.5,-1.1));
#18584=CARTESIAN_POINT('',(2.585,9.5,0.));
#18585=CARTESIAN_POINT('',(2.585,9.5,-1.1));
#18586=CARTESIAN_POINT('Origin',(2.75,9.5,0.));
#18587=CARTESIAN_POINT('Origin',(2.75,9.5,-1.1));
#18588=CARTESIAN_POINT('Origin',(2.75,12.5,-1.1));
#18589=CARTESIAN_POINT('',(2.585,12.5,-1.1));
#18590=CARTESIAN_POINT('Origin',(2.75,12.5,-1.1));
#18591=CARTESIAN_POINT('',(2.585,12.5,0.));
#18592=CARTESIAN_POINT('',(2.585,12.5,-1.1));
#18593=CARTESIAN_POINT('Origin',(2.75,12.5,0.));
#18594=CARTESIAN_POINT('Origin',(2.75,12.5,-1.1));
#18595=CARTESIAN_POINT('Origin',(2.8,-1.,-1.1));
#18596=CARTESIAN_POINT('',(2.635,-1.,-1.1));
#18597=CARTESIAN_POINT('Origin',(2.8,-1.,-1.1));
#18598=CARTESIAN_POINT('',(2.635,-1.,0.));
#18599=CARTESIAN_POINT('',(2.635,-1.,-1.1));
#18600=CARTESIAN_POINT('Origin',(2.8,-1.,0.));
#18601=CARTESIAN_POINT('Origin',(2.8,-1.,-1.1));
#18602=CARTESIAN_POINT('Origin',(-2.8,1.,-1.1));
#18603=CARTESIAN_POINT('',(-2.965,1.,-1.1));
#18604=CARTESIAN_POINT('Origin',(-2.8,1.,-1.1));
#18605=CARTESIAN_POINT('',(-2.965,1.,0.));
#18606=CARTESIAN_POINT('',(-2.965,1.,-1.1));
#18607=CARTESIAN_POINT('Origin',(-2.8,1.,0.));
#18608=CARTESIAN_POINT('Origin',(-2.8,1.,-1.1));
#18609=CARTESIAN_POINT('Origin',(-2.8,-1.,-1.1));
#18610=CARTESIAN_POINT('',(-2.965,-1.,-1.1));
#18611=CARTESIAN_POINT('Origin',(-2.8,-1.,-1.1));
#18612=CARTESIAN_POINT('',(-2.965,-1.,0.));
#18613=CARTESIAN_POINT('',(-2.965,-1.,-1.1));
#18614=CARTESIAN_POINT('Origin',(-2.8,-1.,0.));
#18615=CARTESIAN_POINT('Origin',(-2.8,-1.,-1.1));
#18616=CARTESIAN_POINT('Origin',(2.8,1.,-1.1));
#18617=CARTESIAN_POINT('',(2.635,1.,-1.1));
#18618=CARTESIAN_POINT('Origin',(2.8,1.,-1.1));
#18619=CARTESIAN_POINT('',(2.635,1.,0.));
#18620=CARTESIAN_POINT('',(2.635,1.,-1.1));
#18621=CARTESIAN_POINT('Origin',(2.8,1.,0.));
#18622=CARTESIAN_POINT('Origin',(2.8,1.,-1.1));
#18623=CARTESIAN_POINT('Origin',(18.,0.,-1.1));
#18624=CARTESIAN_POINT('',(17.835,-2.02066721859312E-17,-1.1));
#18625=CARTESIAN_POINT('Origin',(18.,0.,-1.1));
#18626=CARTESIAN_POINT('',(17.835,2.02066721859312E-17,0.));
#18627=CARTESIAN_POINT('',(17.835,-2.02066721859312E-17,-1.1));
#18628=CARTESIAN_POINT('Origin',(18.,0.,0.));
#18629=CARTESIAN_POINT('Origin',(18.,0.,-1.1));
#18630=CARTESIAN_POINT('Origin',(12.,0.,-1.1));
#18631=CARTESIAN_POINT('',(11.835,-2.02066721859312E-17,-1.1));
#18632=CARTESIAN_POINT('Origin',(12.,0.,-1.1));
#18633=CARTESIAN_POINT('',(11.835,2.02066721859312E-17,0.));
#18634=CARTESIAN_POINT('',(11.835,-2.02066721859312E-17,-1.1));
#18635=CARTESIAN_POINT('Origin',(12.,0.,0.));
#18636=CARTESIAN_POINT('Origin',(12.,0.,-1.1));
#18637=CARTESIAN_POINT('Origin',(6.,0.,-1.1));
#18638=CARTESIAN_POINT('',(5.835,-2.02066721859313E-17,-1.1));
#18639=CARTESIAN_POINT('Origin',(6.,0.,-1.1));
#18640=CARTESIAN_POINT('',(5.835,2.02066721859313E-17,0.));
#18641=CARTESIAN_POINT('',(5.835,-2.02066721859313E-17,-1.1));
#18642=CARTESIAN_POINT('Origin',(6.,0.,0.));
#18643=CARTESIAN_POINT('Origin',(6.,0.,-1.1));
#18644=CARTESIAN_POINT('Origin',(24.,0.,-1.1));
#18645=CARTESIAN_POINT('',(23.835,-2.02066721859312E-17,-1.1));
#18646=CARTESIAN_POINT('Origin',(24.,0.,-1.1));
#18647=CARTESIAN_POINT('',(23.835,2.02066721859312E-17,0.));
#18648=CARTESIAN_POINT('',(23.835,-2.02066721859312E-17,-1.1));
#18649=CARTESIAN_POINT('Origin',(24.,0.,0.));
#18650=CARTESIAN_POINT('Origin',(24.,0.,-1.1));
#18651=CARTESIAN_POINT('Origin',(26.,14.,-1.2));
#18652=CARTESIAN_POINT('',(26.,14.,-1.2));
#18653=CARTESIAN_POINT('',(-3.5,14.,-1.2));
#18654=CARTESIAN_POINT('',(26.,14.,-1.2));
#18655=CARTESIAN_POINT('',(-3.5,14.,0.));
#18656=CARTESIAN_POINT('',(-3.5,14.,-1.2));
#18657=CARTESIAN_POINT('',(26.,14.,0.));
#18658=CARTESIAN_POINT('',(26.,14.,0.));
#18659=CARTESIAN_POINT('',(26.,14.,-1.2));
#18660=CARTESIAN_POINT('Origin',(26.,-6.5,-1.2));
#18661=CARTESIAN_POINT('',(26.,-6.5,-1.2));
#18662=CARTESIAN_POINT('',(26.,-6.5,-1.2));
#18663=CARTESIAN_POINT('',(26.,-6.5,0.));
#18664=CARTESIAN_POINT('',(26.,-6.5,0.));
#18665=CARTESIAN_POINT('',(26.,-6.5,-1.2));
#18666=CARTESIAN_POINT('Origin',(-3.5,-6.5,-1.2));
#18667=CARTESIAN_POINT('',(-3.5,-6.5,-1.2));
#18668=CARTESIAN_POINT('',(-3.5,-6.5,-1.2));
#18669=CARTESIAN_POINT('',(-3.5,-6.5,0.));
#18670=CARTESIAN_POINT('',(-3.5,-6.5,0.));
#18671=CARTESIAN_POINT('',(-3.5,-6.5,-1.2));
#18672=CARTESIAN_POINT('Origin',(-3.5,14.,-1.2));
#18673=CARTESIAN_POINT('',(-3.5,14.,-1.2));
#18674=CARTESIAN_POINT('',(-3.5,14.,0.));
#18675=CARTESIAN_POINT('Origin',(11.25,3.75,0.));
#18676=CARTESIAN_POINT('Origin',(11.25,3.75,-1.2));
#23460=UNCERTAINTY_MEASURE_WITH_UNIT(LENGTH_MEASURE(0.001),#23588,
'DISTANCE_ACCURACY_VALUE',
'Maximum model space distance between geometric entities at asserted c
onnectivities');
#23522=UNCERTAINTY_MEASURE_WITH_UNIT(LENGTH_MEASURE(0.001),#23588,
'DISTANCE_ACCURACY_VALUE',
'Maximum model space distance between geometric entities at asserted c
onnectivities');
#23525=(
GEOMETRIC_REPRESENTATION_CONTEXT(3)
GLOBAL_UNCERTAINTY_ASSIGNED_CONTEXT((#23460))
GLOBAL_UNIT_ASSIGNED_CONTEXT((#23588,#23590,#23591))
REPRESENTATION_CONTEXT('','3D')
);
#23587=(
GEOMETRIC_REPRESENTATION_CONTEXT(3)
GLOBAL_UNCERTAINTY_ASSIGNED_CONTEXT((#23522))
GLOBAL_UNIT_ASSIGNED_CONTEXT((#23588,#23590,#23591))
REPRESENTATION_CONTEXT('','3D')
);
#23588=(
LENGTH_UNIT()
NAMED_UNIT(*)
SI_UNIT(.CENTI.,.METRE.)
);
#23590=(
NAMED_UNIT(*)
PLANE_ANGLE_UNIT()
SI_UNIT($,.RADIAN.)
);
#23591=(
NAMED_UNIT(*)
SI_UNIT($,.STERADIAN.)
SOLID_ANGLE_UNIT()
);
#23594=SHAPE_DEFINITION_REPRESENTATION(#23658,#23827);
#23658=PRODUCT_DEFINITION_SHAPE('',$,#23892);
#23827=SHAPE_REPRESENTATION('',(#12878),#23525);
#23889=PRODUCT_DEFINITION_CONTEXT('part definition',#24083,'design');
#23892=PRODUCT_DEFINITION('Base','Base',#23956,#23889);
#23956=PRODUCT_DEFINITION_FORMATION('',$,#24087);
#24083=APPLICATION_CONTEXT(
'Core Data for Automotive Mechanical Design Process');
#24084=PRODUCT_CONTEXT('part definition',#24083,'mechanical');
#24087=PRODUCT('Base','Base','Base',(#24084));
#24184=COLOUR_RGB('Dark Blue',0.08,0.2,0.34);
#24185=FILL_AREA_STYLE_COLOUR('',#24184);
#24186=FILL_AREA_STYLE('',(#24185));
#24187=SURFACE_STYLE_FILL_AREA(#24186);
#24188=SURFACE_SIDE_STYLE('',(#24187));
#24189=SURFACE_STYLE_USAGE(.BOTH.,#24188);
#24190=PRESENTATION_STYLE_ASSIGNMENT((#24189));
ENDSEC;
END-ISO-10303-21;
